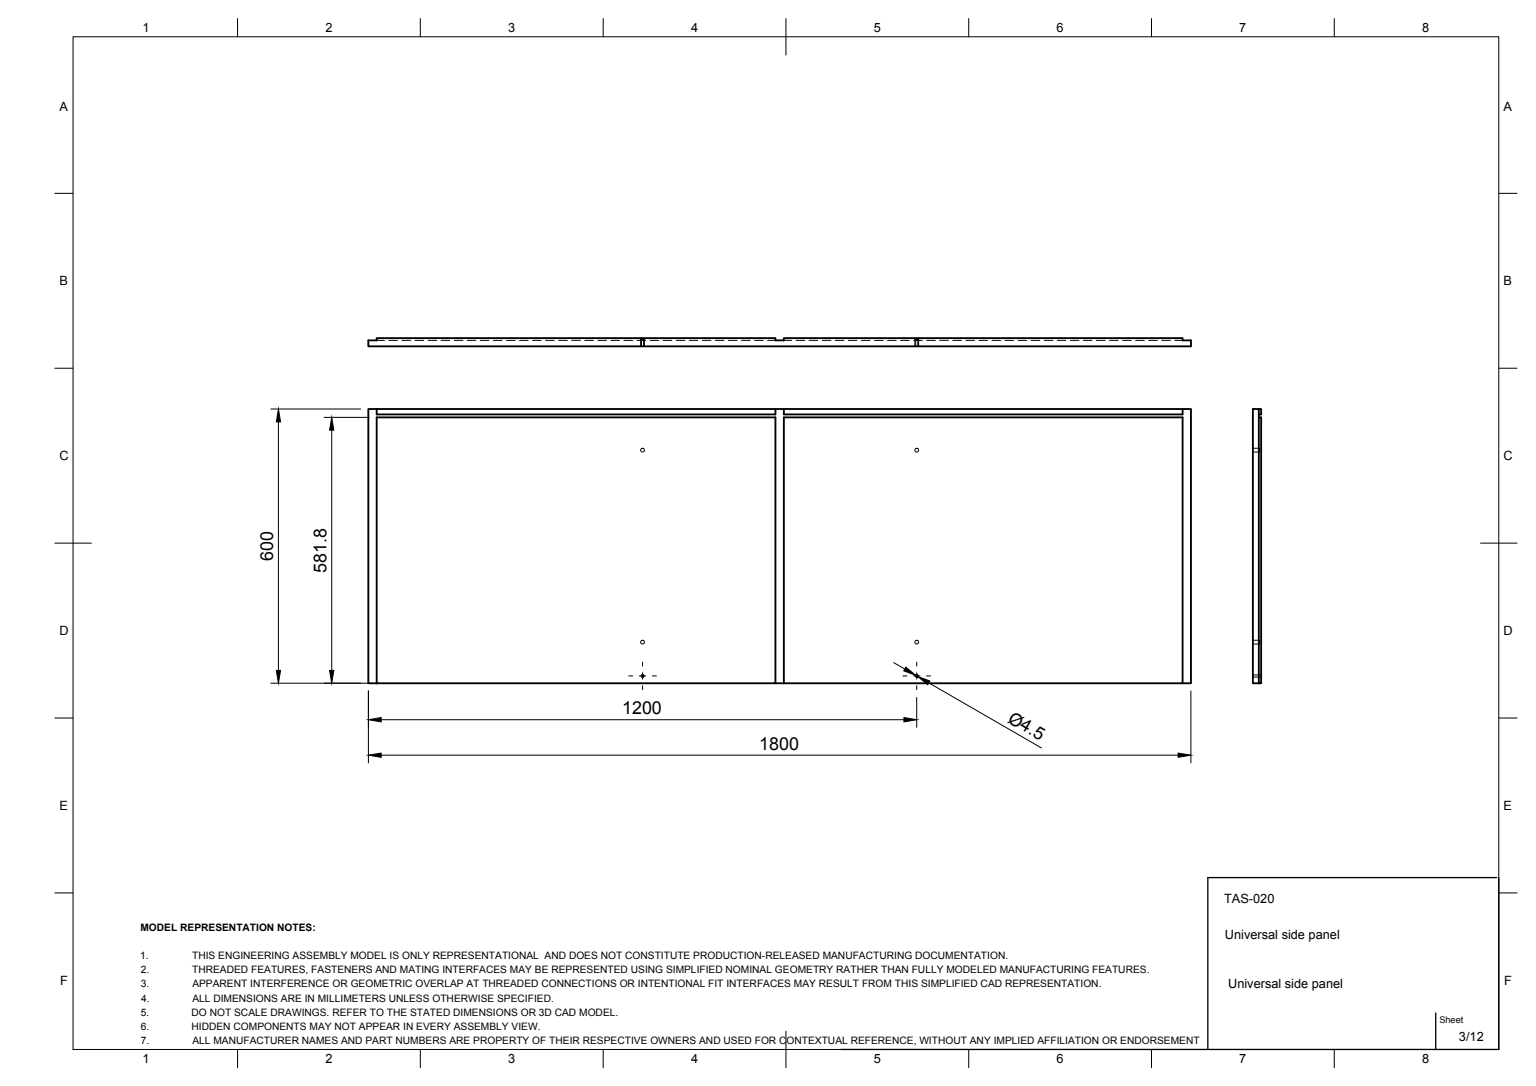
ISO-10303-21;
HEADER;
/* Generated by software containing ST-Developer
 * from STEP Tools, Inc. (www.steptools.com) 
 */

FILE_DESCRIPTION(
/* description */ (''),
/* implementation_level */ '2;1');

FILE_NAME(
/* name */ 'Universal side panel.step',
/* time_stamp */ '2026-11-15T17:46:57-08:00',
/* author */ (''),
/* organization */ (''),
/* preprocessor_version */ 'ST-DEVELOPER v20.2',
/* originating_system */ 'Autodesk Translation Framework v15.17.0.0',
/* authorisation */ '');

FILE_SCHEMA (('AUTOMOTIVE_DESIGN { 1 0 10303 214 3 1 1 }'));
ENDSEC;

DATA;
#10=MECHANICAL_DESIGN_GEOMETRIC_PRESENTATION_REPRESENTATION('',(#376),#12963);
#352=SHAPE_REPRESENTATION_RELATIONSHIP('SRR','None',#13036,#364);
#364=ADVANCED_BREP_SHAPE_REPRESENTATION('',(#388),#12952);
#376=STYLED_ITEM('',(#13105),#388);
#388=MANIFOLD_SOLID_BREP('Body1',#4810);
#409=FACE_BOUND('',#892,.T.);
#410=FACE_BOUND('',#899,.T.);
#411=FACE_BOUND('',#907,.T.);
#412=FACE_BOUND('',#908,.T.);
#413=FACE_BOUND('',#909,.T.);
#414=FACE_BOUND('',#910,.T.);
#415=FACE_BOUND('',#911,.T.);
#416=FACE_BOUND('',#912,.T.);
#469=PLANE('',#5012);
#470=PLANE('',#5016);
#471=PLANE('',#5020);
#472=PLANE('',#5024);
#473=PLANE('',#5031);
#474=PLANE('',#5032);
#475=PLANE('',#5033);
#476=PLANE('',#5034);
#477=PLANE('',#5035);
#478=PLANE('',#5036);
#479=PLANE('',#5037);
#480=PLANE('',#5038);
#481=PLANE('',#5039);
#482=PLANE('',#5040);
#483=PLANE('',#5041);
#484=PLANE('',#5042);
#485=PLANE('',#5043);
#486=PLANE('',#5044);
#487=PLANE('',#5045);
#488=PLANE('',#5046);
#489=PLANE('',#5047);
#490=PLANE('',#5048);
#491=PLANE('',#5049);
#492=PLANE('',#5050);
#493=PLANE('',#5051);
#494=PLANE('',#5052);
#608=FACE_OUTER_BOUND('',#874,.T.);
#609=FACE_OUTER_BOUND('',#875,.T.);
#610=FACE_OUTER_BOUND('',#876,.T.);
#611=FACE_OUTER_BOUND('',#877,.T.);
#612=FACE_OUTER_BOUND('',#878,.T.);
#613=FACE_OUTER_BOUND('',#879,.T.);
#614=FACE_OUTER_BOUND('',#880,.T.);
#615=FACE_OUTER_BOUND('',#881,.T.);
#616=FACE_OUTER_BOUND('',#882,.T.);
#617=FACE_OUTER_BOUND('',#883,.T.);
#618=FACE_OUTER_BOUND('',#884,.T.);
#619=FACE_OUTER_BOUND('',#885,.T.);
#620=FACE_OUTER_BOUND('',#886,.T.);
#621=FACE_OUTER_BOUND('',#887,.T.);
#622=FACE_OUTER_BOUND('',#888,.T.);
#623=FACE_OUTER_BOUND('',#889,.T.);
#624=FACE_OUTER_BOUND('',#890,.T.);
#625=FACE_OUTER_BOUND('',#891,.T.);
#626=FACE_OUTER_BOUND('',#893,.T.);
#627=FACE_OUTER_BOUND('',#894,.T.);
#628=FACE_OUTER_BOUND('',#895,.T.);
#629=FACE_OUTER_BOUND('',#896,.T.);
#630=FACE_OUTER_BOUND('',#897,.T.);
#631=FACE_OUTER_BOUND('',#898,.T.);
#632=FACE_OUTER_BOUND('',#900,.T.);
#633=FACE_OUTER_BOUND('',#901,.T.);
#634=FACE_OUTER_BOUND('',#902,.T.);
#635=FACE_OUTER_BOUND('',#903,.T.);
#636=FACE_OUTER_BOUND('',#904,.T.);
#637=FACE_OUTER_BOUND('',#905,.T.);
#638=FACE_OUTER_BOUND('',#906,.T.);
#639=FACE_OUTER_BOUND('',#913,.T.);
#874=EDGE_LOOP('',(#3280,#3281,#3282,#3283));
#875=EDGE_LOOP('',(#3284));
#876=EDGE_LOOP('',(#3285,#3286,#3287,#3288));
#877=EDGE_LOOP('',(#3289));
#878=EDGE_LOOP('',(#3290,#3291,#3292,#3293));
#879=EDGE_LOOP('',(#3294));
#880=EDGE_LOOP('',(#3295,#3296,#3297,#3298));
#881=EDGE_LOOP('',(#3299));
#882=EDGE_LOOP('',(#3300,#3301,#3302,#3303));
#883=EDGE_LOOP('',(#3304,#3305,#3306,#3307));
#884=EDGE_LOOP('',(#3308,#3309,#3310,#3311));
#885=EDGE_LOOP('',(#3312,#3313,#3314,#3315));
#886=EDGE_LOOP('',(#3316,#3317,#3318,#3319));
#887=EDGE_LOOP('',(#3320,#3321,#3322,#3323));
#888=EDGE_LOOP('',(#3324,#3325,#3326,#3327,#3328,#3329,#3330,#3331,#3332,
#3333,#3334,#3335,#3336,#3337,#3338,#3339,#3340,#3341,#3342,#3343));
#889=EDGE_LOOP('',(#3344,#3345,#3346,#3347));
#890=EDGE_LOOP('',(#3348,#3349,#3350,#3351));
#891=EDGE_LOOP('',(#3352,#3353,#3354,#3355));
#892=EDGE_LOOP('',(#3356));
#893=EDGE_LOOP('',(#3357,#3358,#3359,#3360));
#894=EDGE_LOOP('',(#3361,#3362,#3363,#3364));
#895=EDGE_LOOP('',(#3365,#3366,#3367,#3368));
#896=EDGE_LOOP('',(#3369,#3370,#3371,#3372));
#897=EDGE_LOOP('',(#3373,#3374,#3375,#3376));
#898=EDGE_LOOP('',(#3377,#3378,#3379,#3380));
#899=EDGE_LOOP('',(#3381));
#900=EDGE_LOOP('',(#3382,#3383,#3384,#3385));
#901=EDGE_LOOP('',(#3386,#3387,#3388,#3389));
#902=EDGE_LOOP('',(#3390,#3391,#3392,#3393));
#903=EDGE_LOOP('',(#3394,#3395,#3396,#3397,#3398,#3399,#3400,#3401,#3402,
#3403,#3404,#3405));
#904=EDGE_LOOP('',(#3406,#3407,#3408,#3409));
#905=EDGE_LOOP('',(#3410,#3411,#3412,#3413,#3414,#3415,#3416,#3417,#3418,
#3419,#3420,#3421));
#906=EDGE_LOOP('',(#3422,#3423,#3424,#3425));
#907=EDGE_LOOP('',(#3426));
#908=EDGE_LOOP('',(#3427));
#909=EDGE_LOOP('',(#3428));
#910=EDGE_LOOP('',(#3429));
#911=EDGE_LOOP('',(#3430));
#912=EDGE_LOOP('',(#3431));
#913=EDGE_LOOP('',(#3432,#3433,#3434,#3435));
#1194=LINE('',#6700,#1596);
#1195=LINE('',#6707,#1597);
#1196=LINE('',#6714,#1598);
#1197=LINE('',#6721,#1599);
#1198=LINE('',#6728,#1600);
#1199=LINE('',#6734,#1601);
#1200=LINE('',#6739,#1602);
#1201=LINE('',#6741,#1603);
#1202=LINE('',#6743,#1604);
#1203=LINE('',#6744,#1605);
#1204=LINE('',#6748,#1606);
#1205=LINE('',#6750,#1607);
#1206=LINE('',#6752,#1608);
#1207=LINE('',#6753,#1609);
#1208=LINE('',#6757,#1610);
#1209=LINE('',#6759,#1611);
#1210=LINE('',#6761,#1612);
#1211=LINE('',#6762,#1613);
#1212=LINE('',#6766,#1614);
#1213=LINE('',#6768,#1615);
#1214=LINE('',#6770,#1616);
#1215=LINE('',#6771,#1617);
#1216=LINE('',#6774,#1618);
#1217=LINE('',#6776,#1619);
#1218=LINE('',#6778,#1620);
#1219=LINE('',#6780,#1621);
#1220=LINE('',#6781,#1622);
#1221=LINE('',#6783,#1623);
#1222=LINE('',#6785,#1624);
#1223=LINE('',#6786,#1625);
#1224=LINE('',#6788,#1626);
#1225=LINE('',#6790,#1627);
#1226=LINE('',#6792,#1628);
#1227=LINE('',#6794,#1629);
#1228=LINE('',#6795,#1630);
#1229=LINE('',#6797,#1631);
#1230=LINE('',#6799,#1632);
#1231=LINE('',#6800,#1633);
#1232=LINE('',#6803,#1634);
#1233=LINE('',#6804,#1635);
#1234=LINE('',#6807,#1636);
#1235=LINE('',#6808,#1637);
#1236=LINE('',#6811,#1638);
#1237=LINE('',#6812,#1639);
#1238=LINE('',#6815,#1640);
#1239=LINE('',#6816,#1641);
#1240=LINE('',#6818,#1642);
#1241=LINE('',#6820,#1643);
#1242=LINE('',#6823,#1644);
#1243=LINE('',#6824,#1645);
#1244=LINE('',#6827,#1646);
#1245=LINE('',#6828,#1647);
#1246=LINE('',#6831,#1648);
#1247=LINE('',#6832,#1649);
#1248=LINE('',#6835,#1650);
#1249=LINE('',#6836,#1651);
#1250=LINE('',#6838,#1652);
#1251=LINE('',#6840,#1653);
#1252=LINE('',#6843,#1654);
#1253=LINE('',#6845,#1655);
#1254=LINE('',#6846,#1656);
#1255=LINE('',#6849,#1657);
#1256=LINE('',#6850,#1658);
#1257=LINE('',#6853,#1659);
#1258=LINE('',#6854,#1660);
#1259=LINE('',#6856,#1661);
#1596=VECTOR('',#5523,0.409999999999997);
#1597=VECTOR('',#5532,0.409999999999997);
#1598=VECTOR('',#5541,0.409999999999997);
#1599=VECTOR('',#5550,0.409999999999997);
#1600=VECTOR('',#5559,0.225000000000001);
#1601=VECTOR('',#5566,0.224999999999994);
#1602=VECTOR('',#5571,1.);
#1603=VECTOR('',#5572,1.);
#1604=VECTOR('',#5573,1.);
#1605=VECTOR('',#5574,1.);
#1606=VECTOR('',#5577,1.);
#1607=VECTOR('',#5578,1.);
#1608=VECTOR('',#5579,1.);
#1609=VECTOR('',#5580,1.);
#1610=VECTOR('',#5583,1.);
#1611=VECTOR('',#5584,1.);
#1612=VECTOR('',#5585,1.);
#1613=VECTOR('',#5586,1.);
#1614=VECTOR('',#5589,1.);
#1615=VECTOR('',#5590,1.);
#1616=VECTOR('',#5591,1.);
#1617=VECTOR('',#5592,1.);
#1618=VECTOR('',#5595,1.);
#1619=VECTOR('',#5596,1.);
#1620=VECTOR('',#5597,1.);
#1621=VECTOR('',#5598,1.);
#1622=VECTOR('',#5599,1.);
#1623=VECTOR('',#5600,1.);
#1624=VECTOR('',#5601,1.);
#1625=VECTOR('',#5602,1.);
#1626=VECTOR('',#5603,1.);
#1627=VECTOR('',#5604,1.);
#1628=VECTOR('',#5605,1.);
#1629=VECTOR('',#5606,1.);
#1630=VECTOR('',#5607,1.);
#1631=VECTOR('',#5608,1.);
#1632=VECTOR('',#5609,1.);
#1633=VECTOR('',#5610,1.);
#1634=VECTOR('',#5613,1.);
#1635=VECTOR('',#5614,1.);
#1636=VECTOR('',#5617,1.);
#1637=VECTOR('',#5618,1.);
#1638=VECTOR('',#5621,1.);
#1639=VECTOR('',#5622,1.);
#1640=VECTOR('',#5625,1.);
#1641=VECTOR('',#5626,1.);
#1642=VECTOR('',#5629,1.);
#1643=VECTOR('',#5632,1.);
#1644=VECTOR('',#5635,1.);
#1645=VECTOR('',#5636,1.);
#1646=VECTOR('',#5639,1.);
#1647=VECTOR('',#5640,1.);
#1648=VECTOR('',#5643,1.);
#1649=VECTOR('',#5644,1.);
#1650=VECTOR('',#5647,1.);
#1651=VECTOR('',#5648,1.);
#1652=VECTOR('',#5651,1.);
#1653=VECTOR('',#5654,1.);
#1654=VECTOR('',#5657,1.);
#1655=VECTOR('',#5658,1.);
#1656=VECTOR('',#5659,1.);
#1657=VECTOR('',#5662,1.);
#1658=VECTOR('',#5663,1.);
#1659=VECTOR('',#5666,1.);
#1660=VECTOR('',#5667,1.);
#1661=VECTOR('',#5670,1.);
#1946=CIRCLE('',#5010,0.409999999999997);
#1947=CIRCLE('',#5011,0.409999999999997);
#1948=CIRCLE('',#5014,0.409999999999997);
#1949=CIRCLE('',#5015,0.409999999999997);
#1950=CIRCLE('',#5018,0.409999999999997);
#1951=CIRCLE('',#5019,0.409999999999997);
#1952=CIRCLE('',#5022,0.409999999999997);
#1953=CIRCLE('',#5023,0.409999999999997);
#1954=CIRCLE('',#5026,0.225000000000001);
#1955=CIRCLE('',#5027,0.225000000000001);
#1956=CIRCLE('',#5029,0.224999999999994);
#1957=CIRCLE('',#5030,0.224999999999994);
#2068=VERTEX_POINT('',#6697);
#2069=VERTEX_POINT('',#6699);
#2070=VERTEX_POINT('',#6704);
#2071=VERTEX_POINT('',#6706);
#2072=VERTEX_POINT('',#6711);
#2073=VERTEX_POINT('',#6713);
#2074=VERTEX_POINT('',#6718);
#2075=VERTEX_POINT('',#6720);
#2076=VERTEX_POINT('',#6725);
#2077=VERTEX_POINT('',#6727);
#2078=VERTEX_POINT('',#6731);
#2079=VERTEX_POINT('',#6733);
#2080=VERTEX_POINT('',#6737);
#2081=VERTEX_POINT('',#6738);
#2082=VERTEX_POINT('',#6740);
#2083=VERTEX_POINT('',#6742);
#2084=VERTEX_POINT('',#6746);
#2085=VERTEX_POINT('',#6747);
#2086=VERTEX_POINT('',#6749);
#2087=VERTEX_POINT('',#6751);
#2088=VERTEX_POINT('',#6755);
#2089=VERTEX_POINT('',#6756);
#2090=VERTEX_POINT('',#6758);
#2091=VERTEX_POINT('',#6760);
#2092=VERTEX_POINT('',#6764);
#2093=VERTEX_POINT('',#6765);
#2094=VERTEX_POINT('',#6767);
#2095=VERTEX_POINT('',#6769);
#2096=VERTEX_POINT('',#6773);
#2097=VERTEX_POINT('',#6775);
#2098=VERTEX_POINT('',#6777);
#2099=VERTEX_POINT('',#6779);
#2100=VERTEX_POINT('',#6782);
#2101=VERTEX_POINT('',#6784);
#2102=VERTEX_POINT('',#6787);
#2103=VERTEX_POINT('',#6789);
#2104=VERTEX_POINT('',#6791);
#2105=VERTEX_POINT('',#6793);
#2106=VERTEX_POINT('',#6796);
#2107=VERTEX_POINT('',#6798);
#2108=VERTEX_POINT('',#6802);
#2109=VERTEX_POINT('',#6806);
#2110=VERTEX_POINT('',#6810);
#2111=VERTEX_POINT('',#6814);
#2112=VERTEX_POINT('',#6822);
#2113=VERTEX_POINT('',#6826);
#2114=VERTEX_POINT('',#6830);
#2115=VERTEX_POINT('',#6834);
#2116=VERTEX_POINT('',#6842);
#2117=VERTEX_POINT('',#6844);
#2118=VERTEX_POINT('',#6848);
#2119=VERTEX_POINT('',#6852);
#2536=EDGE_CURVE('',#2068,#2068,#1946,.T.);
#2537=EDGE_CURVE('',#2068,#2069,#1194,.T.);
#2538=EDGE_CURVE('',#2069,#2069,#1947,.T.);
#2539=EDGE_CURVE('',#2070,#2070,#1948,.T.);
#2540=EDGE_CURVE('',#2070,#2071,#1195,.T.);
#2541=EDGE_CURVE('',#2071,#2071,#1949,.T.);
#2542=EDGE_CURVE('',#2072,#2072,#1950,.T.);
#2543=EDGE_CURVE('',#2072,#2073,#1196,.T.);
#2544=EDGE_CURVE('',#2073,#2073,#1951,.T.);
#2545=EDGE_CURVE('',#2074,#2074,#1952,.T.);
#2546=EDGE_CURVE('',#2074,#2075,#1197,.T.);
#2547=EDGE_CURVE('',#2075,#2075,#1953,.T.);
#2548=EDGE_CURVE('',#2076,#2076,#1954,.T.);
#2549=EDGE_CURVE('',#2076,#2077,#1198,.T.);
#2550=EDGE_CURVE('',#2077,#2077,#1955,.T.);
#2551=EDGE_CURVE('',#2078,#2078,#1956,.T.);
#2552=EDGE_CURVE('',#2078,#2079,#1199,.T.);
#2553=EDGE_CURVE('',#2079,#2079,#1957,.T.);
#2554=EDGE_CURVE('',#2080,#2081,#1200,.T.);
#2555=EDGE_CURVE('',#2082,#2080,#1201,.T.);
#2556=EDGE_CURVE('',#2083,#2082,#1202,.T.);
#2557=EDGE_CURVE('',#2081,#2083,#1203,.T.);
#2558=EDGE_CURVE('',#2084,#2085,#1204,.T.);
#2559=EDGE_CURVE('',#2086,#2084,#1205,.T.);
#2560=EDGE_CURVE('',#2087,#2086,#1206,.T.);
#2561=EDGE_CURVE('',#2085,#2087,#1207,.T.);
#2562=EDGE_CURVE('',#2088,#2089,#1208,.T.);
#2563=EDGE_CURVE('',#2090,#2088,#1209,.T.);
#2564=EDGE_CURVE('',#2091,#2090,#1210,.T.);
#2565=EDGE_CURVE('',#2091,#2089,#1211,.T.);
#2566=EDGE_CURVE('',#2092,#2093,#1212,.T.);
#2567=EDGE_CURVE('',#2094,#2092,#1213,.T.);
#2568=EDGE_CURVE('',#2095,#2094,#1214,.T.);
#2569=EDGE_CURVE('',#2095,#2093,#1215,.T.);
#2570=EDGE_CURVE('',#2096,#2084,#1216,.T.);
#2571=EDGE_CURVE('',#2097,#2096,#1217,.T.);
#2572=EDGE_CURVE('',#2098,#2097,#1218,.T.);
#2573=EDGE_CURVE('',#2099,#2098,#1219,.T.);
#2574=EDGE_CURVE('',#2093,#2099,#1220,.T.);
#2575=EDGE_CURVE('',#2095,#2100,#1221,.T.);
#2576=EDGE_CURVE('',#2101,#2100,#1222,.T.);
#2577=EDGE_CURVE('',#2089,#2101,#1223,.T.);
#2578=EDGE_CURVE('',#2091,#2102,#1224,.T.);
#2579=EDGE_CURVE('',#2103,#2102,#1225,.T.);
#2580=EDGE_CURVE('',#2104,#2103,#1226,.T.);
#2581=EDGE_CURVE('',#2105,#2104,#1227,.T.);
#2582=EDGE_CURVE('',#2105,#2082,#1228,.T.);
#2583=EDGE_CURVE('',#2106,#2080,#1229,.T.);
#2584=EDGE_CURVE('',#2107,#2106,#1230,.T.);
#2585=EDGE_CURVE('',#2107,#2086,#1231,.T.);
#2586=EDGE_CURVE('',#2108,#2099,#1232,.T.);
#2587=EDGE_CURVE('',#2092,#2108,#1233,.T.);
#2588=EDGE_CURVE('',#2109,#2085,#1234,.T.);
#2589=EDGE_CURVE('',#2096,#2109,#1235,.T.);
#2590=EDGE_CURVE('',#2110,#2108,#1236,.T.);
#2591=EDGE_CURVE('',#2110,#2094,#1237,.T.);
#2592=EDGE_CURVE('',#2087,#2111,#1238,.T.);
#2593=EDGE_CURVE('',#2111,#2109,#1239,.T.);
#2594=EDGE_CURVE('',#2100,#2110,#1240,.T.);
#2595=EDGE_CURVE('',#2111,#2107,#1241,.T.);
#2596=EDGE_CURVE('',#2112,#2101,#1242,.T.);
#2597=EDGE_CURVE('',#2088,#2112,#1243,.T.);
#2598=EDGE_CURVE('',#2113,#2081,#1244,.T.);
#2599=EDGE_CURVE('',#2106,#2113,#1245,.T.);
#2600=EDGE_CURVE('',#2114,#2112,#1246,.T.);
#2601=EDGE_CURVE('',#2114,#2090,#1247,.T.);
#2602=EDGE_CURVE('',#2083,#2115,#1248,.T.);
#2603=EDGE_CURVE('',#2115,#2113,#1249,.T.);
#2604=EDGE_CURVE('',#2102,#2114,#1250,.T.);
#2605=EDGE_CURVE('',#2115,#2105,#1251,.T.);
#2606=EDGE_CURVE('',#2104,#2116,#1252,.T.);
#2607=EDGE_CURVE('',#2116,#2117,#1253,.T.);
#2608=EDGE_CURVE('',#2097,#2117,#1254,.T.);
#2609=EDGE_CURVE('',#2118,#2103,#1255,.T.);
#2610=EDGE_CURVE('',#2116,#2118,#1256,.T.);
#2611=EDGE_CURVE('',#2119,#2098,#1257,.T.);
#2612=EDGE_CURVE('',#2118,#2119,#1258,.T.);
#2613=EDGE_CURVE('',#2117,#2119,#1259,.T.);
#3280=ORIENTED_EDGE('',*,*,#2536,.F.);
#3281=ORIENTED_EDGE('',*,*,#2537,.T.);
#3282=ORIENTED_EDGE('',*,*,#2538,.T.);
#3283=ORIENTED_EDGE('',*,*,#2537,.F.);
#3284=ORIENTED_EDGE('',*,*,#2538,.F.);
#3285=ORIENTED_EDGE('',*,*,#2539,.F.);
#3286=ORIENTED_EDGE('',*,*,#2540,.T.);
#3287=ORIENTED_EDGE('',*,*,#2541,.T.);
#3288=ORIENTED_EDGE('',*,*,#2540,.F.);
#3289=ORIENTED_EDGE('',*,*,#2541,.F.);
#3290=ORIENTED_EDGE('',*,*,#2542,.F.);
#3291=ORIENTED_EDGE('',*,*,#2543,.T.);
#3292=ORIENTED_EDGE('',*,*,#2544,.T.);
#3293=ORIENTED_EDGE('',*,*,#2543,.F.);
#3294=ORIENTED_EDGE('',*,*,#2544,.F.);
#3295=ORIENTED_EDGE('',*,*,#2545,.F.);
#3296=ORIENTED_EDGE('',*,*,#2546,.T.);
#3297=ORIENTED_EDGE('',*,*,#2547,.T.);
#3298=ORIENTED_EDGE('',*,*,#2546,.F.);
#3299=ORIENTED_EDGE('',*,*,#2547,.F.);
#3300=ORIENTED_EDGE('',*,*,#2548,.F.);
#3301=ORIENTED_EDGE('',*,*,#2549,.T.);
#3302=ORIENTED_EDGE('',*,*,#2550,.F.);
#3303=ORIENTED_EDGE('',*,*,#2549,.F.);
#3304=ORIENTED_EDGE('',*,*,#2551,.F.);
#3305=ORIENTED_EDGE('',*,*,#2552,.T.);
#3306=ORIENTED_EDGE('',*,*,#2553,.F.);
#3307=ORIENTED_EDGE('',*,*,#2552,.F.);
#3308=ORIENTED_EDGE('',*,*,#2554,.F.);
#3309=ORIENTED_EDGE('',*,*,#2555,.F.);
#3310=ORIENTED_EDGE('',*,*,#2556,.F.);
#3311=ORIENTED_EDGE('',*,*,#2557,.F.);
#3312=ORIENTED_EDGE('',*,*,#2558,.F.);
#3313=ORIENTED_EDGE('',*,*,#2559,.F.);
#3314=ORIENTED_EDGE('',*,*,#2560,.F.);
#3315=ORIENTED_EDGE('',*,*,#2561,.F.);
#3316=ORIENTED_EDGE('',*,*,#2562,.F.);
#3317=ORIENTED_EDGE('',*,*,#2563,.F.);
#3318=ORIENTED_EDGE('',*,*,#2564,.F.);
#3319=ORIENTED_EDGE('',*,*,#2565,.T.);
#3320=ORIENTED_EDGE('',*,*,#2566,.F.);
#3321=ORIENTED_EDGE('',*,*,#2567,.F.);
#3322=ORIENTED_EDGE('',*,*,#2568,.F.);
#3323=ORIENTED_EDGE('',*,*,#2569,.T.);
#3324=ORIENTED_EDGE('',*,*,#2570,.F.);
#3325=ORIENTED_EDGE('',*,*,#2571,.F.);
#3326=ORIENTED_EDGE('',*,*,#2572,.F.);
#3327=ORIENTED_EDGE('',*,*,#2573,.F.);
#3328=ORIENTED_EDGE('',*,*,#2574,.F.);
#3329=ORIENTED_EDGE('',*,*,#2569,.F.);
#3330=ORIENTED_EDGE('',*,*,#2575,.T.);
#3331=ORIENTED_EDGE('',*,*,#2576,.F.);
#3332=ORIENTED_EDGE('',*,*,#2577,.F.);
#3333=ORIENTED_EDGE('',*,*,#2565,.F.);
#3334=ORIENTED_EDGE('',*,*,#2578,.T.);
#3335=ORIENTED_EDGE('',*,*,#2579,.F.);
#3336=ORIENTED_EDGE('',*,*,#2580,.F.);
#3337=ORIENTED_EDGE('',*,*,#2581,.F.);
#3338=ORIENTED_EDGE('',*,*,#2582,.T.);
#3339=ORIENTED_EDGE('',*,*,#2555,.T.);
#3340=ORIENTED_EDGE('',*,*,#2583,.F.);
#3341=ORIENTED_EDGE('',*,*,#2584,.F.);
#3342=ORIENTED_EDGE('',*,*,#2585,.T.);
#3343=ORIENTED_EDGE('',*,*,#2559,.T.);
#3344=ORIENTED_EDGE('',*,*,#2566,.T.);
#3345=ORIENTED_EDGE('',*,*,#2574,.T.);
#3346=ORIENTED_EDGE('',*,*,#2586,.F.);
#3347=ORIENTED_EDGE('',*,*,#2587,.F.);
#3348=ORIENTED_EDGE('',*,*,#2558,.T.);
#3349=ORIENTED_EDGE('',*,*,#2588,.F.);
#3350=ORIENTED_EDGE('',*,*,#2589,.F.);
#3351=ORIENTED_EDGE('',*,*,#2570,.T.);
#3352=ORIENTED_EDGE('',*,*,#2567,.T.);
#3353=ORIENTED_EDGE('',*,*,#2587,.T.);
#3354=ORIENTED_EDGE('',*,*,#2590,.F.);
#3355=ORIENTED_EDGE('',*,*,#2591,.T.);
#3356=ORIENTED_EDGE('',*,*,#2551,.T.);
#3357=ORIENTED_EDGE('',*,*,#2561,.T.);
#3358=ORIENTED_EDGE('',*,*,#2592,.T.);
#3359=ORIENTED_EDGE('',*,*,#2593,.T.);
#3360=ORIENTED_EDGE('',*,*,#2588,.T.);
#3361=ORIENTED_EDGE('',*,*,#2568,.T.);
#3362=ORIENTED_EDGE('',*,*,#2591,.F.);
#3363=ORIENTED_EDGE('',*,*,#2594,.F.);
#3364=ORIENTED_EDGE('',*,*,#2575,.F.);
#3365=ORIENTED_EDGE('',*,*,#2560,.T.);
#3366=ORIENTED_EDGE('',*,*,#2585,.F.);
#3367=ORIENTED_EDGE('',*,*,#2595,.F.);
#3368=ORIENTED_EDGE('',*,*,#2592,.F.);
#3369=ORIENTED_EDGE('',*,*,#2562,.T.);
#3370=ORIENTED_EDGE('',*,*,#2577,.T.);
#3371=ORIENTED_EDGE('',*,*,#2596,.F.);
#3372=ORIENTED_EDGE('',*,*,#2597,.F.);
#3373=ORIENTED_EDGE('',*,*,#2554,.T.);
#3374=ORIENTED_EDGE('',*,*,#2598,.F.);
#3375=ORIENTED_EDGE('',*,*,#2599,.F.);
#3376=ORIENTED_EDGE('',*,*,#2583,.T.);
#3377=ORIENTED_EDGE('',*,*,#2563,.T.);
#3378=ORIENTED_EDGE('',*,*,#2597,.T.);
#3379=ORIENTED_EDGE('',*,*,#2600,.F.);
#3380=ORIENTED_EDGE('',*,*,#2601,.T.);
#3381=ORIENTED_EDGE('',*,*,#2548,.T.);
#3382=ORIENTED_EDGE('',*,*,#2557,.T.);
#3383=ORIENTED_EDGE('',*,*,#2602,.T.);
#3384=ORIENTED_EDGE('',*,*,#2603,.T.);
#3385=ORIENTED_EDGE('',*,*,#2598,.T.);
#3386=ORIENTED_EDGE('',*,*,#2564,.T.);
#3387=ORIENTED_EDGE('',*,*,#2601,.F.);
#3388=ORIENTED_EDGE('',*,*,#2604,.F.);
#3389=ORIENTED_EDGE('',*,*,#2578,.F.);
#3390=ORIENTED_EDGE('',*,*,#2556,.T.);
#3391=ORIENTED_EDGE('',*,*,#2582,.F.);
#3392=ORIENTED_EDGE('',*,*,#2605,.F.);
#3393=ORIENTED_EDGE('',*,*,#2602,.F.);
#3394=ORIENTED_EDGE('',*,*,#2595,.T.);
#3395=ORIENTED_EDGE('',*,*,#2584,.T.);
#3396=ORIENTED_EDGE('',*,*,#2599,.T.);
#3397=ORIENTED_EDGE('',*,*,#2603,.F.);
#3398=ORIENTED_EDGE('',*,*,#2605,.T.);
#3399=ORIENTED_EDGE('',*,*,#2581,.T.);
#3400=ORIENTED_EDGE('',*,*,#2606,.T.);
#3401=ORIENTED_EDGE('',*,*,#2607,.T.);
#3402=ORIENTED_EDGE('',*,*,#2608,.F.);
#3403=ORIENTED_EDGE('',*,*,#2571,.T.);
#3404=ORIENTED_EDGE('',*,*,#2589,.T.);
#3405=ORIENTED_EDGE('',*,*,#2593,.F.);
#3406=ORIENTED_EDGE('',*,*,#2580,.T.);
#3407=ORIENTED_EDGE('',*,*,#2609,.F.);
#3408=ORIENTED_EDGE('',*,*,#2610,.F.);
#3409=ORIENTED_EDGE('',*,*,#2606,.F.);
#3410=ORIENTED_EDGE('',*,*,#2594,.T.);
#3411=ORIENTED_EDGE('',*,*,#2590,.T.);
#3412=ORIENTED_EDGE('',*,*,#2586,.T.);
#3413=ORIENTED_EDGE('',*,*,#2573,.T.);
#3414=ORIENTED_EDGE('',*,*,#2611,.F.);
#3415=ORIENTED_EDGE('',*,*,#2612,.F.);
#3416=ORIENTED_EDGE('',*,*,#2609,.T.);
#3417=ORIENTED_EDGE('',*,*,#2579,.T.);
#3418=ORIENTED_EDGE('',*,*,#2604,.T.);
#3419=ORIENTED_EDGE('',*,*,#2600,.T.);
#3420=ORIENTED_EDGE('',*,*,#2596,.T.);
#3421=ORIENTED_EDGE('',*,*,#2576,.T.);
#3422=ORIENTED_EDGE('',*,*,#2610,.T.);
#3423=ORIENTED_EDGE('',*,*,#2612,.T.);
#3424=ORIENTED_EDGE('',*,*,#2613,.F.);
#3425=ORIENTED_EDGE('',*,*,#2607,.F.);
#3426=ORIENTED_EDGE('',*,*,#2553,.T.);
#3427=ORIENTED_EDGE('',*,*,#2550,.T.);
#3428=ORIENTED_EDGE('',*,*,#2545,.T.);
#3429=ORIENTED_EDGE('',*,*,#2542,.T.);
#3430=ORIENTED_EDGE('',*,*,#2539,.T.);
#3431=ORIENTED_EDGE('',*,*,#2536,.T.);
#3432=ORIENTED_EDGE('',*,*,#2572,.T.);
#3433=ORIENTED_EDGE('',*,*,#2608,.T.);
#3434=ORIENTED_EDGE('',*,*,#2613,.T.);
#3435=ORIENTED_EDGE('',*,*,#2611,.T.);
#4440=CYLINDRICAL_SURFACE('',#5009,0.409999999999997);
#4441=CYLINDRICAL_SURFACE('',#5013,0.409999999999997);
#4442=CYLINDRICAL_SURFACE('',#5017,0.409999999999997);
#4443=CYLINDRICAL_SURFACE('',#5021,0.409999999999997);
#4444=CYLINDRICAL_SURFACE('',#5025,0.225000000000001);
#4445=CYLINDRICAL_SURFACE('',#5028,0.224999999999994);
#4589=ADVANCED_FACE('',(#608),#4440,.F.);
#4590=ADVANCED_FACE('',(#609),#469,.F.);
#4591=ADVANCED_FACE('',(#610),#4441,.F.);
#4592=ADVANCED_FACE('',(#611),#470,.F.);
#4593=ADVANCED_FACE('',(#612),#4442,.F.);
#4594=ADVANCED_FACE('',(#613),#471,.F.);
#4595=ADVANCED_FACE('',(#614),#4443,.F.);
#4596=ADVANCED_FACE('',(#615),#472,.F.);
#4597=ADVANCED_FACE('',(#616),#4444,.F.);
#4598=ADVANCED_FACE('',(#617),#4445,.F.);
#4599=ADVANCED_FACE('',(#618),#473,.F.);
#4600=ADVANCED_FACE('',(#619),#474,.F.);
#4601=ADVANCED_FACE('',(#620),#475,.F.);
#4602=ADVANCED_FACE('',(#621),#476,.F.);
#4603=ADVANCED_FACE('',(#622),#477,.F.);
#4604=ADVANCED_FACE('',(#623),#478,.T.);
#4605=ADVANCED_FACE('',(#624),#479,.T.);
#4606=ADVANCED_FACE('',(#625,#409),#480,.T.);
#4607=ADVANCED_FACE('',(#626),#481,.T.);
#4608=ADVANCED_FACE('',(#627),#482,.F.);
#4609=ADVANCED_FACE('',(#628),#483,.F.);
#4610=ADVANCED_FACE('',(#629),#484,.T.);
#4611=ADVANCED_FACE('',(#630),#485,.T.);
#4612=ADVANCED_FACE('',(#631,#410),#486,.T.);
#4613=ADVANCED_FACE('',(#632),#487,.T.);
#4614=ADVANCED_FACE('',(#633),#488,.F.);
#4615=ADVANCED_FACE('',(#634),#489,.F.);
#4616=ADVANCED_FACE('',(#635),#490,.T.);
#4617=ADVANCED_FACE('',(#636),#491,.F.);
#4618=ADVANCED_FACE('',(#637),#492,.T.);
#4619=ADVANCED_FACE('',(#638,#411,#412,#413,#414,#415,#416),#493,.T.);
#4620=ADVANCED_FACE('',(#639),#494,.T.);
#4810=CLOSED_SHELL('',(#4589,#4590,#4591,#4592,#4593,#4594,#4595,#4596,
#4597,#4598,#4599,#4600,#4601,#4602,#4603,#4604,#4605,#4606,#4607,#4608,
#4609,#4610,#4611,#4612,#4613,#4614,#4615,#4616,#4617,#4618,#4619,#4620));
#5008=AXIS2_PLACEMENT_3D('',#6695,#5517,#5518);
#5009=AXIS2_PLACEMENT_3D('',#6696,#5519,#5520);
#5010=AXIS2_PLACEMENT_3D('',#6698,#5521,#5522);
#5011=AXIS2_PLACEMENT_3D('',#6701,#5524,#5525);
#5012=AXIS2_PLACEMENT_3D('',#6702,#5526,#5527);
#5013=AXIS2_PLACEMENT_3D('',#6703,#5528,#5529);
#5014=AXIS2_PLACEMENT_3D('',#6705,#5530,#5531);
#5015=AXIS2_PLACEMENT_3D('',#6708,#5533,#5534);
#5016=AXIS2_PLACEMENT_3D('',#6709,#5535,#5536);
#5017=AXIS2_PLACEMENT_3D('',#6710,#5537,#5538);
#5018=AXIS2_PLACEMENT_3D('',#6712,#5539,#5540);
#5019=AXIS2_PLACEMENT_3D('',#6715,#5542,#5543);
#5020=AXIS2_PLACEMENT_3D('',#6716,#5544,#5545);
#5021=AXIS2_PLACEMENT_3D('',#6717,#5546,#5547);
#5022=AXIS2_PLACEMENT_3D('',#6719,#5548,#5549);
#5023=AXIS2_PLACEMENT_3D('',#6722,#5551,#5552);
#5024=AXIS2_PLACEMENT_3D('',#6723,#5553,#5554);
#5025=AXIS2_PLACEMENT_3D('',#6724,#5555,#5556);
#5026=AXIS2_PLACEMENT_3D('',#6726,#5557,#5558);
#5027=AXIS2_PLACEMENT_3D('',#6729,#5560,#5561);
#5028=AXIS2_PLACEMENT_3D('',#6730,#5562,#5563);
#5029=AXIS2_PLACEMENT_3D('',#6732,#5564,#5565);
#5030=AXIS2_PLACEMENT_3D('',#6735,#5567,#5568);
#5031=AXIS2_PLACEMENT_3D('',#6736,#5569,#5570);
#5032=AXIS2_PLACEMENT_3D('',#6745,#5575,#5576);
#5033=AXIS2_PLACEMENT_3D('',#6754,#5581,#5582);
#5034=AXIS2_PLACEMENT_3D('',#6763,#5587,#5588);
#5035=AXIS2_PLACEMENT_3D('',#6772,#5593,#5594);
#5036=AXIS2_PLACEMENT_3D('',#6801,#5611,#5612);
#5037=AXIS2_PLACEMENT_3D('',#6805,#5615,#5616);
#5038=AXIS2_PLACEMENT_3D('',#6809,#5619,#5620);
#5039=AXIS2_PLACEMENT_3D('',#6813,#5623,#5624);
#5040=AXIS2_PLACEMENT_3D('',#6817,#5627,#5628);
#5041=AXIS2_PLACEMENT_3D('',#6819,#5630,#5631);
#5042=AXIS2_PLACEMENT_3D('',#6821,#5633,#5634);
#5043=AXIS2_PLACEMENT_3D('',#6825,#5637,#5638);
#5044=AXIS2_PLACEMENT_3D('',#6829,#5641,#5642);
#5045=AXIS2_PLACEMENT_3D('',#6833,#5645,#5646);
#5046=AXIS2_PLACEMENT_3D('',#6837,#5649,#5650);
#5047=AXIS2_PLACEMENT_3D('',#6839,#5652,#5653);
#5048=AXIS2_PLACEMENT_3D('',#6841,#5655,#5656);
#5049=AXIS2_PLACEMENT_3D('',#6847,#5660,#5661);
#5050=AXIS2_PLACEMENT_3D('',#6851,#5664,#5665);
#5051=AXIS2_PLACEMENT_3D('',#6855,#5668,#5669);
#5052=AXIS2_PLACEMENT_3D('',#6857,#5671,#5672);
#5517=DIRECTION('axis',(0.,0.,1.));
#5518=DIRECTION('refdir',(1.,0.,0.));
#5519=DIRECTION('center_axis',(1.,0.,0.));
#5520=DIRECTION('ref_axis',(0.,0.,-1.));
#5521=DIRECTION('center_axis',(1.,0.,0.));
#5522=DIRECTION('ref_axis',(0.,0.,-1.));
#5523=DIRECTION('',(1.,0.,0.));
#5524=DIRECTION('center_axis',(1.,0.,0.));
#5525=DIRECTION('ref_axis',(0.,0.,-1.));
#5526=DIRECTION('center_axis',(1.,0.,0.));
#5527=DIRECTION('ref_axis',(0.,0.,-1.));
#5528=DIRECTION('center_axis',(1.,0.,0.));
#5529=DIRECTION('ref_axis',(0.,0.,-1.));
#5530=DIRECTION('center_axis',(1.,0.,0.));
#5531=DIRECTION('ref_axis',(0.,0.,-1.));
#5532=DIRECTION('',(1.,0.,0.));
#5533=DIRECTION('center_axis',(1.,0.,0.));
#5534=DIRECTION('ref_axis',(0.,0.,-1.));
#5535=DIRECTION('center_axis',(1.,0.,0.));
#5536=DIRECTION('ref_axis',(0.,0.,-1.));
#5537=DIRECTION('center_axis',(1.,0.,0.));
#5538=DIRECTION('ref_axis',(0.,0.,-1.));
#5539=DIRECTION('center_axis',(1.,0.,0.));
#5540=DIRECTION('ref_axis',(0.,0.,-1.));
#5541=DIRECTION('',(1.,0.,0.));
#5542=DIRECTION('center_axis',(1.,0.,0.));
#5543=DIRECTION('ref_axis',(0.,0.,-1.));
#5544=DIRECTION('center_axis',(1.,0.,0.));
#5545=DIRECTION('ref_axis',(0.,0.,-1.));
#5546=DIRECTION('center_axis',(1.,0.,0.));
#5547=DIRECTION('ref_axis',(0.,0.,-1.));
#5548=DIRECTION('center_axis',(1.,0.,0.));
#5549=DIRECTION('ref_axis',(0.,0.,-1.));
#5550=DIRECTION('',(1.,0.,0.));
#5551=DIRECTION('center_axis',(1.,0.,0.));
#5552=DIRECTION('ref_axis',(0.,0.,-1.));
#5553=DIRECTION('center_axis',(1.,0.,0.));
#5554=DIRECTION('ref_axis',(0.,0.,-1.));
#5555=DIRECTION('center_axis',(-1.,0.,0.));
#5556=DIRECTION('ref_axis',(0.,0.,-1.));
#5557=DIRECTION('center_axis',(-1.,0.,0.));
#5558=DIRECTION('ref_axis',(0.,0.,-1.));
#5559=DIRECTION('',(-1.,0.,0.));
#5560=DIRECTION('center_axis',(1.,0.,0.));
#5561=DIRECTION('ref_axis',(0.,0.,-1.));
#5562=DIRECTION('center_axis',(-1.,0.,0.));
#5563=DIRECTION('ref_axis',(0.,0.,-1.));
#5564=DIRECTION('center_axis',(-1.,0.,0.));
#5565=DIRECTION('ref_axis',(0.,0.,-1.));
#5566=DIRECTION('',(-1.,0.,0.));
#5567=DIRECTION('center_axis',(1.,0.,0.));
#5568=DIRECTION('ref_axis',(0.,0.,-1.));
#5569=DIRECTION('center_axis',(0.,1.,0.));
#5570=DIRECTION('ref_axis',(-1.,0.,0.));
#5571=DIRECTION('',(1.,0.,0.));
#5572=DIRECTION('',(0.,0.,1.));
#5573=DIRECTION('',(-1.,0.,0.));
#5574=DIRECTION('',(0.,0.,-1.));
#5575=DIRECTION('center_axis',(0.,1.,0.));
#5576=DIRECTION('ref_axis',(-1.,0.,0.));
#5577=DIRECTION('',(1.,0.,0.));
#5578=DIRECTION('',(0.,0.,1.));
#5579=DIRECTION('',(-1.,0.,0.));
#5580=DIRECTION('',(0.,0.,-1.));
#5581=DIRECTION('center_axis',(0.,-1.,0.));
#5582=DIRECTION('ref_axis',(1.,0.,0.));
#5583=DIRECTION('',(-1.,0.,0.));
#5584=DIRECTION('',(0.,0.,1.));
#5585=DIRECTION('',(1.,0.,0.));
#5586=DIRECTION('',(0.,0.,1.));
#5587=DIRECTION('center_axis',(0.,-1.,0.));
#5588=DIRECTION('ref_axis',(1.,0.,0.));
#5589=DIRECTION('',(-1.,0.,0.));
#5590=DIRECTION('',(0.,0.,1.));
#5591=DIRECTION('',(1.,0.,0.));
#5592=DIRECTION('',(0.,0.,1.));
#5593=DIRECTION('center_axis',(-1.,0.,0.));
#5594=DIRECTION('ref_axis',(0.,-1.,0.));
#5595=DIRECTION('',(0.,-1.,0.));
#5596=DIRECTION('',(0.,0.,-1.));
#5597=DIRECTION('',(0.,1.,0.));
#5598=DIRECTION('',(0.,0.,1.));
#5599=DIRECTION('',(0.,-1.,0.));
#5600=DIRECTION('',(0.,-1.,0.));
#5601=DIRECTION('',(0.,0.,1.));
#5602=DIRECTION('',(0.,-1.,0.));
#5603=DIRECTION('',(0.,-1.,0.));
#5604=DIRECTION('',(0.,0.,1.));
#5605=DIRECTION('',(0.,-1.,0.));
#5606=DIRECTION('',(0.,0.,-1.));
#5607=DIRECTION('',(0.,-1.,0.));
#5608=DIRECTION('',(0.,-1.,0.));
#5609=DIRECTION('',(0.,0.,-1.));
#5610=DIRECTION('',(0.,-1.,0.));
#5611=DIRECTION('center_axis',(0.,0.,1.));
#5612=DIRECTION('ref_axis',(1.,0.,0.));
#5613=DIRECTION('',(-1.,0.,0.));
#5614=DIRECTION('',(0.,-1.,0.));
#5615=DIRECTION('center_axis',(0.,0.,1.));
#5616=DIRECTION('ref_axis',(1.,0.,0.));
#5617=DIRECTION('',(0.,-1.,0.));
#5618=DIRECTION('',(1.,0.,0.));
#5619=DIRECTION('center_axis',(1.,0.,0.));
#5620=DIRECTION('ref_axis',(0.,1.,0.));
#5621=DIRECTION('',(0.,0.,1.));
#5622=DIRECTION('',(0.,1.,0.));
#5623=DIRECTION('center_axis',(1.,0.,0.));
#5624=DIRECTION('ref_axis',(0.,1.,0.));
#5625=DIRECTION('',(0.,1.,0.));
#5626=DIRECTION('',(0.,0.,1.));
#5627=DIRECTION('center_axis',(0.,0.,1.));
#5628=DIRECTION('ref_axis',(1.,0.,0.));
#5629=DIRECTION('',(1.,0.,0.));
#5630=DIRECTION('center_axis',(0.,0.,1.));
#5631=DIRECTION('ref_axis',(1.,0.,0.));
#5632=DIRECTION('',(-1.,0.,0.));
#5633=DIRECTION('center_axis',(0.,0.,1.));
#5634=DIRECTION('ref_axis',(1.,0.,0.));
#5635=DIRECTION('',(-1.,0.,0.));
#5636=DIRECTION('',(0.,-1.,0.));
#5637=DIRECTION('center_axis',(0.,0.,1.));
#5638=DIRECTION('ref_axis',(1.,0.,0.));
#5639=DIRECTION('',(0.,-1.,0.));
#5640=DIRECTION('',(1.,0.,0.));
#5641=DIRECTION('center_axis',(1.,0.,0.));
#5642=DIRECTION('ref_axis',(0.,1.,0.));
#5643=DIRECTION('',(0.,0.,1.));
#5644=DIRECTION('',(0.,1.,0.));
#5645=DIRECTION('center_axis',(1.,0.,0.));
#5646=DIRECTION('ref_axis',(0.,1.,0.));
#5647=DIRECTION('',(0.,1.,0.));
#5648=DIRECTION('',(0.,0.,1.));
#5649=DIRECTION('center_axis',(0.,0.,1.));
#5650=DIRECTION('ref_axis',(1.,0.,0.));
#5651=DIRECTION('',(1.,0.,0.));
#5652=DIRECTION('center_axis',(0.,0.,1.));
#5653=DIRECTION('ref_axis',(1.,0.,0.));
#5654=DIRECTION('',(-1.,0.,0.));
#5655=DIRECTION('center_axis',(0.,1.,0.));
#5656=DIRECTION('ref_axis',(-1.,0.,0.));
#5657=DIRECTION('',(-1.,0.,0.));
#5658=DIRECTION('',(0.,0.,1.));
#5659=DIRECTION('',(-1.,0.,0.));
#5660=DIRECTION('center_axis',(0.,0.,1.));
#5661=DIRECTION('ref_axis',(1.,0.,0.));
#5662=DIRECTION('',(1.,0.,0.));
#5663=DIRECTION('',(0.,-1.,0.));
#5664=DIRECTION('center_axis',(0.,-1.,0.));
#5665=DIRECTION('ref_axis',(1.,0.,0.));
#5666=DIRECTION('',(1.,0.,0.));
#5667=DIRECTION('',(0.,0.,1.));
#5668=DIRECTION('center_axis',(-1.,0.,0.));
#5669=DIRECTION('ref_axis',(0.,-1.,0.));
#5670=DIRECTION('',(0.,-1.,0.));
#5671=DIRECTION('center_axis',(0.,0.,1.));
#5672=DIRECTION('ref_axis',(1.,0.,0.));
#6695=CARTESIAN_POINT('',(0.,0.,0.));
#6696=CARTESIAN_POINT('Origin',(0.,51.,60.));
#6697=CARTESIAN_POINT('',(0.,51.,60.41));
#6698=CARTESIAN_POINT('Origin',(0.,51.,60.));
#6699=CARTESIAN_POINT('',(1.5,51.,60.41));
#6700=CARTESIAN_POINT('',(0.,51.,60.41));
#6701=CARTESIAN_POINT('Origin',(1.5,51.,60.));
#6702=CARTESIAN_POINT('Origin',(1.5,51.,60.));
#6703=CARTESIAN_POINT('Origin',(0.,9.,120.));
#6704=CARTESIAN_POINT('',(0.,9.,120.41));
#6705=CARTESIAN_POINT('Origin',(0.,9.,120.));
#6706=CARTESIAN_POINT('',(1.5,9.,120.41));
#6707=CARTESIAN_POINT('',(0.,9.,120.41));
#6708=CARTESIAN_POINT('Origin',(1.5,9.,120.));
#6709=CARTESIAN_POINT('Origin',(1.5,9.,120.));
#6710=CARTESIAN_POINT('Origin',(0.,9.,60.));
#6711=CARTESIAN_POINT('',(0.,9.,60.41));
#6712=CARTESIAN_POINT('Origin',(0.,9.,60.));
#6713=CARTESIAN_POINT('',(1.5,9.,60.41));
#6714=CARTESIAN_POINT('',(0.,9.,60.41));
#6715=CARTESIAN_POINT('Origin',(1.5,9.,60.));
#6716=CARTESIAN_POINT('Origin',(1.5,9.,60.));
#6717=CARTESIAN_POINT('Origin',(0.,51.,120.));
#6718=CARTESIAN_POINT('',(0.,51.,120.41));
#6719=CARTESIAN_POINT('Origin',(0.,51.,120.));
#6720=CARTESIAN_POINT('',(1.5,51.,120.41));
#6721=CARTESIAN_POINT('',(0.,51.,120.41));
#6722=CARTESIAN_POINT('Origin',(1.5,51.,120.));
#6723=CARTESIAN_POINT('Origin',(1.5,51.,120.));
#6724=CARTESIAN_POINT('Origin',(1.8,1.6,60.));
#6725=CARTESIAN_POINT('',(1.8,1.6,60.225));
#6726=CARTESIAN_POINT('Origin',(1.8,1.6,60.));
#6727=CARTESIAN_POINT('',(0.,1.6,60.225));
#6728=CARTESIAN_POINT('',(1.8,1.6,60.225));
#6729=CARTESIAN_POINT('Origin',(0.,1.6,60.));
#6730=CARTESIAN_POINT('Origin',(1.8,1.6,120.));
#6731=CARTESIAN_POINT('',(1.8,1.6,120.225));
#6732=CARTESIAN_POINT('Origin',(1.8,1.6,120.));
#6733=CARTESIAN_POINT('',(0.,1.6,120.225));
#6734=CARTESIAN_POINT('',(1.8,1.6,120.225));
#6735=CARTESIAN_POINT('Origin',(0.,1.6,120.));
#6736=CARTESIAN_POINT('Origin',(1.81,58.82,0.));
#6737=CARTESIAN_POINT('',(1.3,58.82,89.08));
#6738=CARTESIAN_POINT('',(1.8,58.82,89.08));
#6739=CARTESIAN_POINT('',(1.6825,58.82,89.08));
#6740=CARTESIAN_POINT('',(1.3,58.82,1.82));
#6741=CARTESIAN_POINT('',(1.3,58.82,0.));
#6742=CARTESIAN_POINT('',(1.8,58.82,1.82));
#6743=CARTESIAN_POINT('',(1.6825,58.82,1.82));
#6744=CARTESIAN_POINT('',(1.8,58.82,0.));
#6745=CARTESIAN_POINT('Origin',(1.81,58.82,0.));
#6746=CARTESIAN_POINT('',(1.3,58.82,178.18));
#6747=CARTESIAN_POINT('',(1.8,58.82,178.18));
#6748=CARTESIAN_POINT('',(1.6825,58.82,178.18));
#6749=CARTESIAN_POINT('',(1.3,58.82,90.92));
#6750=CARTESIAN_POINT('',(1.3,58.82,0.));
#6751=CARTESIAN_POINT('',(1.8,58.82,90.92));
#6752=CARTESIAN_POINT('',(1.6825,58.82,90.92));
#6753=CARTESIAN_POINT('',(1.8,58.82,0.));
#6754=CARTESIAN_POINT('Origin',(1.3,58.18,0.));
#6755=CARTESIAN_POINT('',(1.8,58.18,89.08));
#6756=CARTESIAN_POINT('',(1.3,58.18,89.08));
#6757=CARTESIAN_POINT('',(1.4275,58.18,89.08));
#6758=CARTESIAN_POINT('',(1.8,58.18,1.82));
#6759=CARTESIAN_POINT('',(1.8,58.18,0.));
#6760=CARTESIAN_POINT('',(1.3,58.18,1.82));
#6761=CARTESIAN_POINT('',(1.4275,58.18,1.82));
#6762=CARTESIAN_POINT('',(1.3,58.18,0.));
#6763=CARTESIAN_POINT('Origin',(1.3,58.18,0.));
#6764=CARTESIAN_POINT('',(1.8,58.18,178.18));
#6765=CARTESIAN_POINT('',(1.3,58.18,178.18));
#6766=CARTESIAN_POINT('',(1.4275,58.18,178.18));
#6767=CARTESIAN_POINT('',(1.8,58.18,90.92));
#6768=CARTESIAN_POINT('',(1.8,58.18,0.));
#6769=CARTESIAN_POINT('',(1.3,58.18,90.92));
#6770=CARTESIAN_POINT('',(1.4275,58.18,90.92));
#6771=CARTESIAN_POINT('',(1.3,58.18,0.));
#6772=CARTESIAN_POINT('Origin',(1.3,60.,178.18));
#6773=CARTESIAN_POINT('',(1.3,60.,178.18));
#6774=CARTESIAN_POINT('',(1.3,60.,178.18));
#6775=CARTESIAN_POINT('',(1.3,60.,180.));
#6776=CARTESIAN_POINT('',(1.3,60.,89.09));
#6777=CARTESIAN_POINT('',(1.3,0.,180.));
#6778=CARTESIAN_POINT('',(1.3,45.,180.));
#6779=CARTESIAN_POINT('',(1.3,0.,178.18));
#6780=CARTESIAN_POINT('',(1.3,0.,89.09));
#6781=CARTESIAN_POINT('',(1.3,60.,178.18));
#6782=CARTESIAN_POINT('',(1.3,0.,90.92));
#6783=CARTESIAN_POINT('',(1.3,60.,90.92));
#6784=CARTESIAN_POINT('',(1.3,0.,89.08));
#6785=CARTESIAN_POINT('',(1.3,0.,44.54));
#6786=CARTESIAN_POINT('',(1.3,60.,89.08));
#6787=CARTESIAN_POINT('',(1.3,0.,1.82));
#6788=CARTESIAN_POINT('',(1.3,60.,1.82));
#6789=CARTESIAN_POINT('',(1.3,0.,0.));
#6790=CARTESIAN_POINT('',(1.3,0.,0.));
#6791=CARTESIAN_POINT('',(1.3,60.,0.));
#6792=CARTESIAN_POINT('',(1.3,45.,0.));
#6793=CARTESIAN_POINT('',(1.3,60.,1.82));
#6794=CARTESIAN_POINT('',(1.3,60.,0.));
#6795=CARTESIAN_POINT('',(1.3,60.,1.82));
#6796=CARTESIAN_POINT('',(1.3,60.,89.08));
#6797=CARTESIAN_POINT('',(1.3,60.,89.08));
#6798=CARTESIAN_POINT('',(1.3,60.,90.92));
#6799=CARTESIAN_POINT('',(1.3,60.,44.54));
#6800=CARTESIAN_POINT('',(1.3,60.,90.92));
#6801=CARTESIAN_POINT('Origin',(1.555,30.,178.18));
#6802=CARTESIAN_POINT('',(1.8,0.,178.18));
#6803=CARTESIAN_POINT('',(0.7775,0.,178.18));
#6804=CARTESIAN_POINT('',(1.8,15.,178.18));
#6805=CARTESIAN_POINT('Origin',(1.555,30.,178.18));
#6806=CARTESIAN_POINT('',(1.8,60.,178.18));
#6807=CARTESIAN_POINT('',(1.8,15.,178.18));
#6808=CARTESIAN_POINT('',(1.6775,60.,178.18));
#6809=CARTESIAN_POINT('Origin',(1.8,0.,0.));
#6810=CARTESIAN_POINT('',(1.8,0.,90.92));
#6811=CARTESIAN_POINT('',(1.8,0.,0.));
#6812=CARTESIAN_POINT('',(1.8,15.,90.92));
#6813=CARTESIAN_POINT('Origin',(1.8,0.,0.));
#6814=CARTESIAN_POINT('',(1.8,60.,90.92));
#6815=CARTESIAN_POINT('',(1.8,15.,90.92));
#6816=CARTESIAN_POINT('',(1.8,60.,0.));
#6817=CARTESIAN_POINT('Origin',(1.555,30.,90.92));
#6818=CARTESIAN_POINT('',(0.7775,0.,90.92));
#6819=CARTESIAN_POINT('Origin',(1.555,30.,90.92));
#6820=CARTESIAN_POINT('',(1.6775,60.,90.92));
#6821=CARTESIAN_POINT('Origin',(1.555,30.,89.08));
#6822=CARTESIAN_POINT('',(1.8,0.,89.08));
#6823=CARTESIAN_POINT('',(0.7775,0.,89.08));
#6824=CARTESIAN_POINT('',(1.8,15.,89.08));
#6825=CARTESIAN_POINT('Origin',(1.555,30.,89.08));
#6826=CARTESIAN_POINT('',(1.8,60.,89.08));
#6827=CARTESIAN_POINT('',(1.8,15.,89.08));
#6828=CARTESIAN_POINT('',(1.6775,60.,89.08));
#6829=CARTESIAN_POINT('Origin',(1.8,0.,0.));
#6830=CARTESIAN_POINT('',(1.8,0.,1.82));
#6831=CARTESIAN_POINT('',(1.8,0.,0.));
#6832=CARTESIAN_POINT('',(1.8,15.,1.82));
#6833=CARTESIAN_POINT('Origin',(1.8,0.,0.));
#6834=CARTESIAN_POINT('',(1.8,60.,1.82));
#6835=CARTESIAN_POINT('',(1.8,15.,1.82));
#6836=CARTESIAN_POINT('',(1.8,60.,0.));
#6837=CARTESIAN_POINT('Origin',(1.555,30.,1.82));
#6838=CARTESIAN_POINT('',(0.7775,0.,1.82));
#6839=CARTESIAN_POINT('Origin',(1.555,30.,1.82));
#6840=CARTESIAN_POINT('',(1.6775,60.,1.82));
#6841=CARTESIAN_POINT('Origin',(1.8,60.,0.));
#6842=CARTESIAN_POINT('',(0.,60.,0.));
#6843=CARTESIAN_POINT('',(1.8,60.,0.));
#6844=CARTESIAN_POINT('',(0.,60.,180.));
#6845=CARTESIAN_POINT('',(0.,60.,0.));
#6846=CARTESIAN_POINT('',(1.8,60.,180.));
#6847=CARTESIAN_POINT('Origin',(0.9,30.,0.));
#6848=CARTESIAN_POINT('',(0.,0.,0.));
#6849=CARTESIAN_POINT('',(0.,0.,0.));
#6850=CARTESIAN_POINT('',(0.,60.,0.));
#6851=CARTESIAN_POINT('Origin',(0.,0.,0.));
#6852=CARTESIAN_POINT('',(0.,0.,180.));
#6853=CARTESIAN_POINT('',(0.,0.,180.));
#6854=CARTESIAN_POINT('',(0.,0.,0.));
#6855=CARTESIAN_POINT('Origin',(0.,60.,0.));
#6856=CARTESIAN_POINT('',(0.,60.,180.));
#6857=CARTESIAN_POINT('Origin',(0.9,30.,180.));
#12938=UNCERTAINTY_MEASURE_WITH_UNIT(LENGTH_MEASURE(0.001),#12964,
'DISTANCE_ACCURACY_VALUE',
'Maximum model space distance between geometric entities at asserted c
onnectivities');
#12949=UNCERTAINTY_MEASURE_WITH_UNIT(LENGTH_MEASURE(0.001),#12964,
'DISTANCE_ACCURACY_VALUE',
'Maximum model space distance between geometric entities at asserted c
onnectivities');
#12952=(
GEOMETRIC_REPRESENTATION_CONTEXT(3)
GLOBAL_UNCERTAINTY_ASSIGNED_CONTEXT((#12938))
GLOBAL_UNIT_ASSIGNED_CONTEXT((#12964,#12966,#12967))
REPRESENTATION_CONTEXT('','3D')
);
#12963=(
GEOMETRIC_REPRESENTATION_CONTEXT(3)
GLOBAL_UNCERTAINTY_ASSIGNED_CONTEXT((#12949))
GLOBAL_UNIT_ASSIGNED_CONTEXT((#12964,#12966,#12967))
REPRESENTATION_CONTEXT('','3D')
);
#12964=(
LENGTH_UNIT()
NAMED_UNIT(*)
SI_UNIT(.CENTI.,.METRE.)
);
#12966=(
NAMED_UNIT(*)
PLANE_ANGLE_UNIT()
SI_UNIT($,.RADIAN.)
);
#12967=(
NAMED_UNIT(*)
SI_UNIT($,.STERADIAN.)
SOLID_ANGLE_UNIT()
);
#12970=SHAPE_DEFINITION_REPRESENTATION(#12983,#13036);
#12983=PRODUCT_DEFINITION_SHAPE('',$,#13050);
#13036=SHAPE_REPRESENTATION('',(#5008),#12952);
#13047=PRODUCT_DEFINITION_CONTEXT('part definition',#13088,'design');
#13050=PRODUCT_DEFINITION('Universal side panel','Universal side panel',
#13063,#13047);
#13063=PRODUCT_DEFINITION_FORMATION('',$,#13092);
#13088=APPLICATION_CONTEXT(
'Core Data for Automotive Mechanical Design Process');
#13089=PRODUCT_CONTEXT('part definition',#13088,'mechanical');
#13092=PRODUCT('Universal side panel','Universal side panel',$,(#13089));
#13105=PRESENTATION_STYLE_ASSIGNMENT((#13118));
#13118=SURFACE_STYLE_USAGE(.BOTH.,#13131);
#13131=SURFACE_SIDE_STYLE('',(#13144));
#13144=SURFACE_STYLE_FILL_AREA(#13157);
#13157=FILL_AREA_STYLE('Universal side panel finish',(#13170));
#13170=FILL_AREA_STYLE_COLOUR('Universal side panel finish',#13183);
#13183=COLOUR_RGB('Universal side panel finish',0.0941176470588235,0.231372549019608,
0.431372549019608);
ENDSEC;
END-ISO-10303-21;
